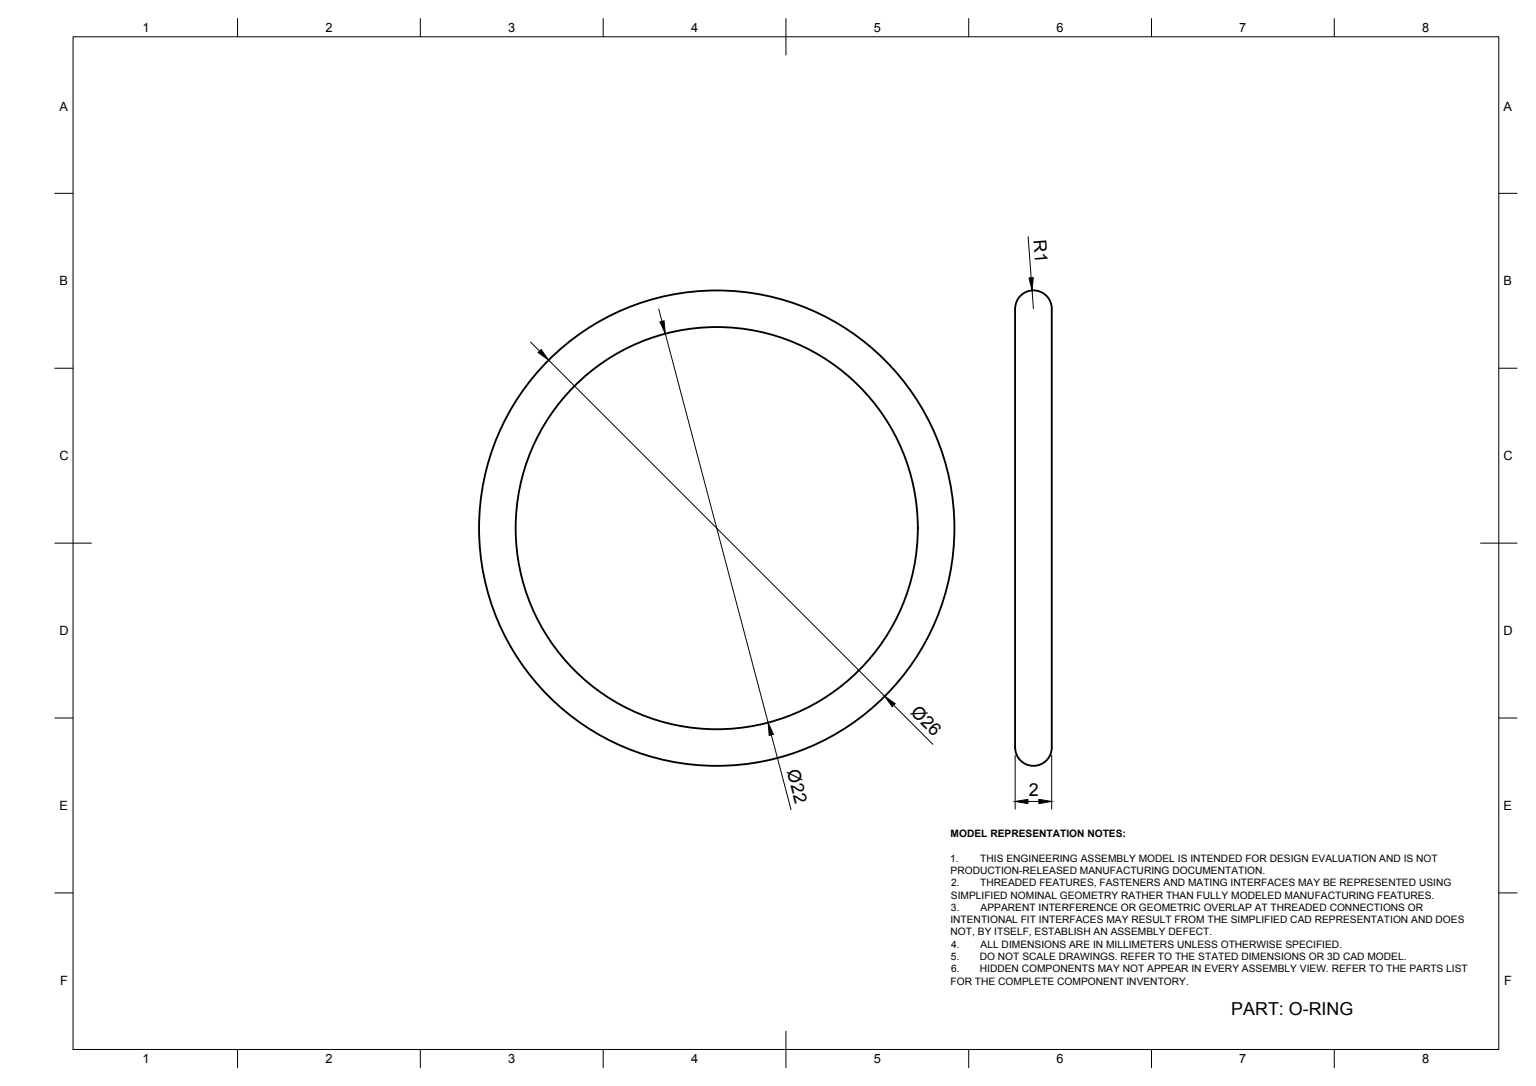
ISO-10303-21;
HEADER;
/* Generated by software containing ST-Developer
 * from STEP Tools, Inc. (www.steptools.com) 
 */

FILE_DESCRIPTION(
/* description */ (''),
/* implementation_level */ '2;1');

FILE_NAME(
/* name */ 'O_Ring.step',
/* time_stamp */ '2026-10-04T22:47:03-07:00',
/* author */ (''),
/* organization */ (''),
/* preprocessor_version */ 'ST-DEVELOPER v20.2',
/* originating_system */ 'Autodesk Translation Framework v15.15.0.0',
/* authorisation */ '');

FILE_SCHEMA (('AUTOMOTIVE_DESIGN { 1 0 10303 214 3 1 1 }'));
ENDSEC;

DATA;
#10=MECHANICAL_DESIGN_GEOMETRIC_PRESENTATION_REPRESENTATION('',(#83),#19878);
#56=TOROIDAL_SURFACE('',#5417,12.,1.);
#69=SHAPE_REPRESENTATION_RELATIONSHIP('SRR','None',#19913,#76);
#76=ADVANCED_BREP_SHAPE_REPRESENTATION('',(#90),#19877);
#83=STYLED_ITEM('',(#19955),#90);
#90=MANIFOLD_SOLID_BREP('Body1',#4831);
#600=FACE_OUTER_BOUND('',#896,.T.);
#896=EDGE_LOOP('',(#4427,#4428,#4429,#4430));
#1873=CIRCLE('',#5418,1.);
#1874=CIRCLE('',#5419,11.);
#2324=VERTEX_POINT('',#19851);
#3025=EDGE_CURVE('',#2324,#2324,#1873,.T.);
#3026=EDGE_CURVE('',#2324,#2324,#1874,.T.);
#4427=ORIENTED_EDGE('',*,*,#3025,.F.);
#4428=ORIENTED_EDGE('',*,*,#3026,.T.);
#4429=ORIENTED_EDGE('',*,*,#3025,.T.);
#4430=ORIENTED_EDGE('',*,*,#3026,.F.);
#4824=ADVANCED_FACE('',(#600),#56,.T.);
#4831=CLOSED_SHELL('',(#4824));
#5416=AXIS2_PLACEMENT_3D('',#19849,#6795,#6796);
#5417=AXIS2_PLACEMENT_3D('',#19850,#6797,#6798);
#5418=AXIS2_PLACEMENT_3D('',#19852,#6799,#6800);
#5419=AXIS2_PLACEMENT_3D('',#19853,#6801,#6802);
#6795=DIRECTION('axis',(0.,0.,1.));
#6796=DIRECTION('refdir',(1.,0.,0.));
#6797=DIRECTION('center_axis',(0.,0.,1.));
#6798=DIRECTION('ref_axis',(1.,0.,0.));
#6799=DIRECTION('center_axis',(1.22464679914735E-16,-1.,0.));
#6800=DIRECTION('ref_axis',(-1.,-1.22464679914735E-16,0.));
#6801=DIRECTION('center_axis',(0.,0.,-1.));
#6802=DIRECTION('ref_axis',(1.,0.,0.));
#19849=CARTESIAN_POINT('',(0.,0.,0.));
#19850=CARTESIAN_POINT('Origin',(0.,0.,-6.72261291411212));
#19851=CARTESIAN_POINT('',(-11.,-1.34711147906209E-15,-6.72261291411212));
#19852=CARTESIAN_POINT('Origin',(-12.,-1.46957615897682E-15,-6.72261291411212));
#19853=CARTESIAN_POINT('Origin',(0.,0.,-6.72261291411212));
#19868=UNCERTAINTY_MEASURE_WITH_UNIT(LENGTH_MEASURE(0.01),#19879,
'DISTANCE_ACCURACY_VALUE',
'Maximum model space distance between geometric entities at asserted c
onnectivities');
#19869=UNCERTAINTY_MEASURE_WITH_UNIT(LENGTH_MEASURE(0.01),#19879,
'DISTANCE_ACCURACY_VALUE',
'Maximum model space distance between geometric entities at asserted c
onnectivities');
#19877=(
GEOMETRIC_REPRESENTATION_CONTEXT(3)
GLOBAL_UNCERTAINTY_ASSIGNED_CONTEXT((#19868))
GLOBAL_UNIT_ASSIGNED_CONTEXT((#19879,#19881,#19882))
REPRESENTATION_CONTEXT('','3D')
);
#19878=(
GEOMETRIC_REPRESENTATION_CONTEXT(3)
GLOBAL_UNCERTAINTY_ASSIGNED_CONTEXT((#19869))
GLOBAL_UNIT_ASSIGNED_CONTEXT((#19879,#19881,#19882))
REPRESENTATION_CONTEXT('','3D')
);
#19879=(
LENGTH_UNIT()
NAMED_UNIT(*)
SI_UNIT(.MILLI.,.METRE.)
);
#19881=(
NAMED_UNIT(*)
PLANE_ANGLE_UNIT()
SI_UNIT($,.RADIAN.)
);
#19882=(
NAMED_UNIT(*)
SI_UNIT($,.STERADIAN.)
SOLID_ANGLE_UNIT()
);
#19890=SHAPE_DEFINITION_REPRESENTATION(#19898,#19913);
#19898=PRODUCT_DEFINITION_SHAPE('',$,#19922);
#19913=SHAPE_REPRESENTATION('',(#5416),#19877);
#19914=PRODUCT_DEFINITION_CONTEXT('part definition',#19940,'design');
#19922=PRODUCT_DEFINITION('O_Ring','O_Ring',#19930,#19914);
#19930=PRODUCT_DEFINITION_FORMATION('',$,#19949);
#19940=APPLICATION_CONTEXT(
'Core Data for Automotive Mechanical Design Process');
#19941=PRODUCT_CONTEXT('part definition',#19940,'mechanical');
#19949=PRODUCT('O_Ring','O_Ring',$,(#19941));
#19955=PRESENTATION_STYLE_ASSIGNMENT((#19961));
#19961=SURFACE_STYLE_USAGE(.BOTH.,#19967);
#19967=SURFACE_SIDE_STYLE('',(#19973));
#19973=SURFACE_STYLE_FILL_AREA(#19979);
#19979=FILL_AREA_STYLE('Opaque(39,39,39)',(#19985));
#19985=FILL_AREA_STYLE_COLOUR('Opaque(39,39,39)',#19991);
#19991=COLOUR_RGB('Opaque(39,39,39)', 0.09019608, 0.27058824, 0.51372549);
ENDSEC;
END-ISO-10303-21;
